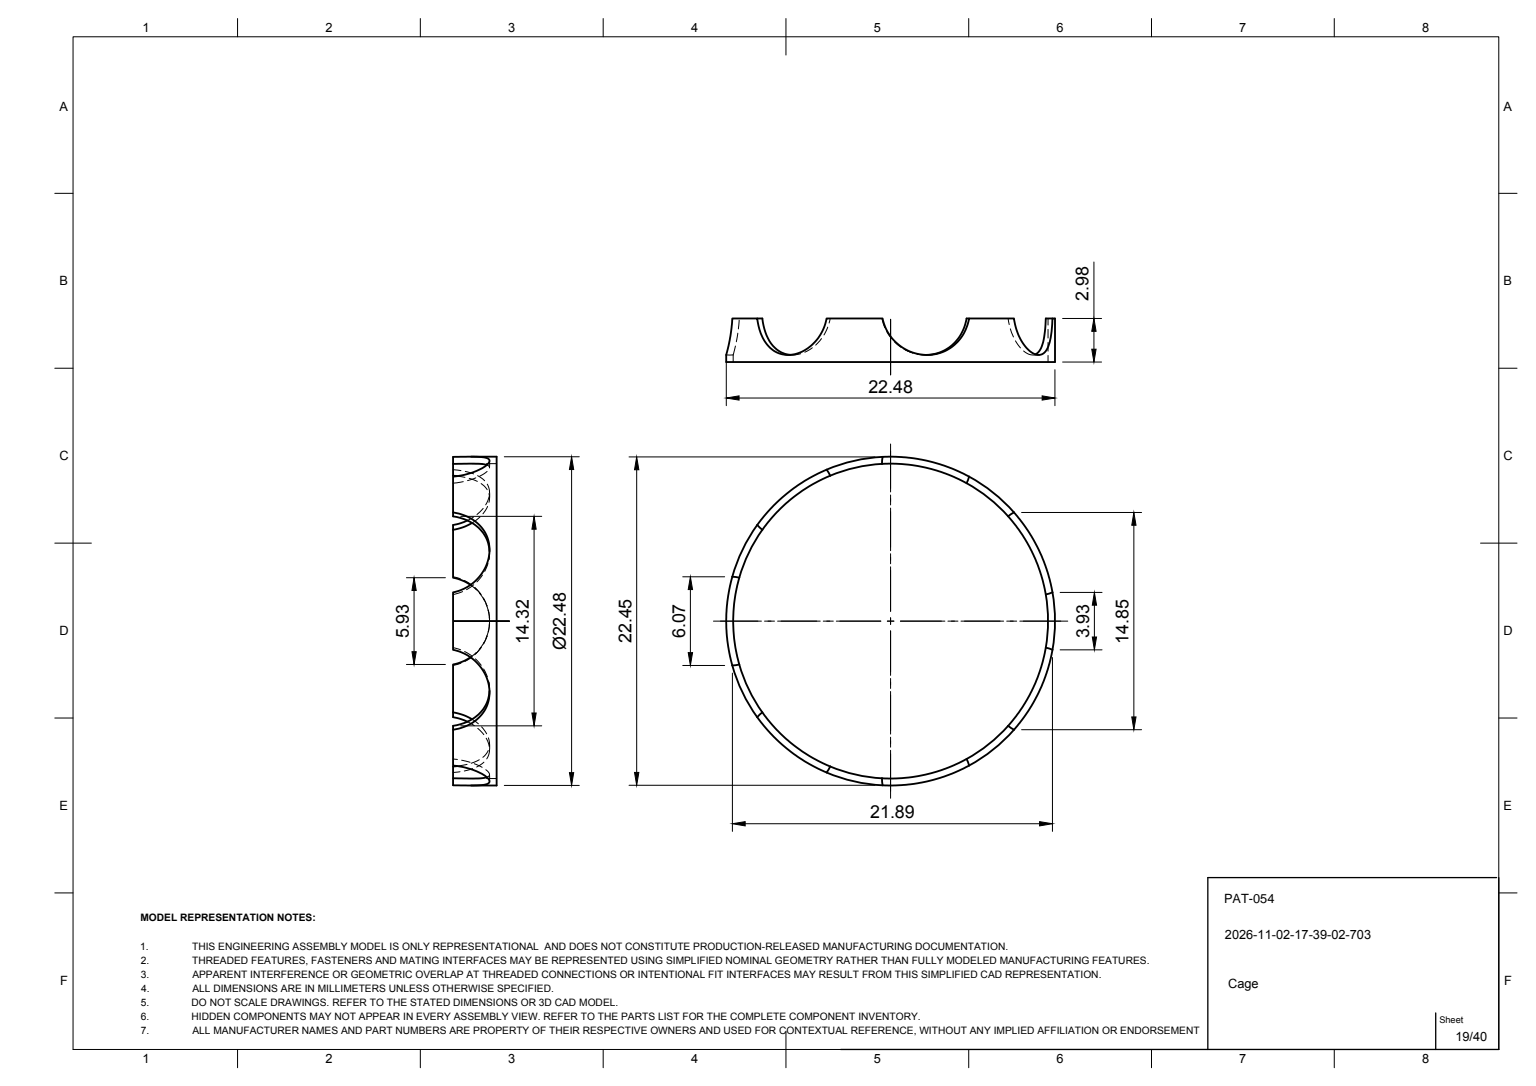
ISO-10303-21;
HEADER;
/* Generated by software containing ST-Developer
 * from STEP Tools, Inc. (www.steptools.com) 
 */

FILE_DESCRIPTION(
/* description */ ('PAT-054'),
/* implementation_level */ '2;1');

FILE_NAME(
/* name */ 'Cage.step',
/* time_stamp */ '2026-10-29T16:38:13-07:00',
/* author */ (''),
/* organization */ (''),
/* preprocessor_version */ 'ST-DEVELOPER v20.2',
/* originating_system */ 'Autodesk Translation Framework v15.17.0.0',
/* authorisation */ '');

FILE_SCHEMA (('AUTOMOTIVE_DESIGN { 1 0 10303 214 3 1 1 }'));
ENDSEC;

DATA;
#10=MECHANICAL_DESIGN_GEOMETRIC_PRESENTATION_REPRESENTATION('',(#917),#33981);
#403=B_SPLINE_CURVE_WITH_KNOTS('',3,(#19369,#19370,#19371,#19372,#19373,
#19374,#19375,#19376,#19377,#19378,#19379,#19380,#19381,#19382,#19383,#19384,
#19385,#19386,#19387,#19388,#19389,#19390),.UNSPECIFIED.,.F.,.F.,(4,2,2,
2,2,2,2,2,2,2,4),(0.0591825211272536,0.157966726598481,0.236950089897721,
0.315933453196962,0.391576304923761,0.46721915665056,0.54286200837736,0.618504860104159,
0.697488223403399,0.77647158670264,0.875255792173867),.UNSPECIFIED.);
#404=B_SPLINE_CURVE_WITH_KNOTS('',3,(#19394,#19395,#19396,#19397,#19398,
#19399,#19400,#19401,#19402,#19403,#19404,#19405,#19406,#19407,#19408,#19409,
#19410,#19411,#19412,#19413,#19414,#19415),.UNSPECIFIED.,.F.,.F.,(4,2,2,
2,2,2,2,2,2,2,4),(0.0581119756758434,0.106553146291161,0.213106292582322,
0.30849933801665,0.386091982889075,0.4636846277615,0.541277272633925,0.61886991750635,
0.714262962940678,0.820816109231839,0.869257279847157),.UNSPECIFIED.);
#405=B_SPLINE_CURVE_WITH_KNOTS('',3,(#19421,#19422,#19423,#19424,#19425,
#19426,#19427,#19428,#19429,#19430,#19431,#19432,#19433,#19434,#19435,#19436,
#19437,#19438,#19439,#19440,#19441,#19442),.UNSPECIFIED.,.F.,.F.,(4,2,2,
2,2,2,2,2,2,2,4),(0.0581119756758434,0.106553146291161,0.213106292582322,
0.30849933801665,0.386091982889075,0.4636846277615,0.541277272633925,0.61886991750635,
0.714262962940679,0.820816109231839,0.869257279847157),.UNSPECIFIED.);
#406=B_SPLINE_CURVE_WITH_KNOTS('',3,(#19446,#19447,#19448,#19449,#19450,
#19451,#19452,#19453,#19454,#19455,#19456,#19457,#19458,#19459,#19460,#19461,
#19462,#19463,#19464,#19465,#19466,#19467),.UNSPECIFIED.,.F.,.F.,(4,2,2,
2,2,2,2,2,2,2,4),(0.0581119756758433,0.106553146291161,0.213106292582322,
0.308499338016649,0.386091982889075,0.4636846277615,0.541277272633925,0.61886991750635,
0.714262962940678,0.820816109231839,0.869257279847157),.UNSPECIFIED.);
#407=B_SPLINE_CURVE_WITH_KNOTS('',3,(#19476,#19477,#19478,#19479,#19480,
#19481,#19482,#19483,#19484,#19485,#19486,#19487,#19488,#19489,#19490,#19491,
#19492,#19493,#19494,#19495,#19496,#19497),.UNSPECIFIED.,.F.,.F.,(4,2,2,
2,2,2,2,2,2,2,4),(0.0581119756758433,0.106553146291161,0.213106292582322,
0.30849933801665,0.386091982889075,0.4636846277615,0.541277272633925,0.61886991750635,
0.714262962940678,0.820816109231839,0.869257279847157),.UNSPECIFIED.);
#408=B_SPLINE_CURVE_WITH_KNOTS('',3,(#19501,#19502,#19503,#19504,#19505,
#19506,#19507,#19508,#19509,#19510,#19511,#19512,#19513,#19514,#19515,#19516,
#19517,#19518,#19519,#19520,#19521,#19522),.UNSPECIFIED.,.F.,.F.,(4,2,2,
2,2,2,2,2,2,2,4),(0.0581119756758434,0.106553146291161,0.213106292582322,
0.30849933801665,0.386091982889075,0.4636846277615,0.541277272633925,0.61886991750635,
0.714262962940678,0.820816109231839,0.869257279847157),.UNSPECIFIED.);
#409=B_SPLINE_CURVE_WITH_KNOTS('',3,(#19526,#19527,#19528,#19529,#19530,
#19531,#19532,#19533,#19534,#19535,#19536,#19537,#19538,#19539,#19540,#19541,
#19542,#19543,#19544,#19545,#19546,#19547),.UNSPECIFIED.,.F.,.F.,(4,2,2,
2,2,2,2,2,2,2,4),(0.0581119756758434,0.106553146291161,0.213106292582322,
0.30849933801665,0.386091982889075,0.4636846277615,0.541277272633925,0.61886991750635,
0.714262962940678,0.820816109231839,0.869257279847157),.UNSPECIFIED.);
#410=B_SPLINE_CURVE_WITH_KNOTS('',3,(#19551,#19552,#19553,#19554,#19555,
#19556,#19557,#19558,#19559,#19560,#19561,#19562,#19563,#19564,#19565,#19566,
#19567,#19568,#19569,#19570,#19571,#19572),.UNSPECIFIED.,.F.,.F.,(4,2,2,
2,2,2,2,2,2,2,4),(0.0581119756758433,0.106553146291161,0.213106292582322,
0.30849933801665,0.386091982889075,0.4636846277615,0.541277272633925,0.61886991750635,
0.714262962940678,0.820816109231839,0.869257279847157),.UNSPECIFIED.);
#411=B_SPLINE_CURVE_WITH_KNOTS('',3,(#19580,#19581,#19582,#19583,#19584,
#19585,#19586,#19587,#19588,#19589,#19590,#19591,#19592,#19593,#19594,#19595,
#19596,#19597,#19598,#19599,#19600,#19601),.UNSPECIFIED.,.F.,.F.,(4,2,2,
2,2,2,2,2,2,2,4),(0.0591825211272536,0.157966726598481,0.236950089897721,
0.315933453196962,0.391576304923761,0.467219156650561,0.54286200837736,
0.618504860104159,0.697488223403399,0.77647158670264,0.875255792173867),
 .UNSPECIFIED.);
#412=B_SPLINE_CURVE_WITH_KNOTS('',3,(#19609,#19610,#19611,#19612,#19613,
#19614,#19615,#19616,#19617,#19618,#19619,#19620,#19621,#19622,#19623,#19624,
#19625,#19626,#19627,#19628,#19629,#19630),.UNSPECIFIED.,.F.,.F.,(4,2,2,
2,2,2,2,2,2,2,4),(0.0591825211272536,0.157966726598481,0.236950089897722,
0.315933453196962,0.391576304923761,0.467219156650561,0.54286200837736,
0.618504860104159,0.697488223403399,0.77647158670264,0.875255792173867),
 .UNSPECIFIED.);
#413=B_SPLINE_CURVE_WITH_KNOTS('',3,(#19640,#19641,#19642,#19643,#19644,
#19645,#19646,#19647,#19648,#19649,#19650,#19651,#19652,#19653,#19654,#19655,
#19656,#19657,#19658,#19659,#19660,#19661),.UNSPECIFIED.,.F.,.F.,(4,2,2,
2,2,2,2,2,2,2,4),(0.0591825211272536,0.157966726598481,0.236950089897721,
0.315933453196962,0.391576304923761,0.46721915665056,0.54286200837736,0.618504860104159,
0.697488223403399,0.77647158670264,0.875255792173867),.UNSPECIFIED.);
#414=B_SPLINE_CURVE_WITH_KNOTS('',3,(#19669,#19670,#19671,#19672,#19673,
#19674,#19675,#19676,#19677,#19678,#19679,#19680,#19681,#19682,#19683,#19684,
#19685,#19686,#19687,#19688,#19689,#19690),.UNSPECIFIED.,.F.,.F.,(4,2,2,
2,2,2,2,2,2,2,4),(0.0591825211272536,0.157966726598481,0.236950089897721,
0.315933453196962,0.391576304923761,0.46721915665056,0.542862008377359,
0.618504860104159,0.697488223403399,0.776471586702639,0.875255792173867),
 .UNSPECIFIED.);
#415=B_SPLINE_CURVE_WITH_KNOTS('',3,(#19698,#19699,#19700,#19701,#19702,
#19703,#19704,#19705,#19706,#19707,#19708,#19709,#19710,#19711,#19712,#19713,
#19714,#19715,#19716,#19717,#19718,#19719),.UNSPECIFIED.,.F.,.F.,(4,2,2,
2,2,2,2,2,2,2,4),(0.0591825211272536,0.157966726598481,0.236950089897721,
0.315933453196962,0.391576304923761,0.46721915665056,0.54286200837736,0.618504860104159,
0.697488223403399,0.77647158670264,0.875255792173867),.UNSPECIFIED.);
#416=B_SPLINE_CURVE_WITH_KNOTS('',3,(#19728,#19729,#19730,#19731,#19732,
#19733,#19734,#19735,#19736,#19737,#19738,#19739,#19740,#19741,#19742,#19743,
#19744,#19745,#19746,#19747,#19748,#19749),.UNSPECIFIED.,.F.,.F.,(4,2,2,
2,2,2,2,2,2,2,4),(0.0591825211272536,0.157966726598481,0.236950089897721,
0.315933453196962,0.391576304923761,0.46721915665056,0.542862008377359,
0.618504860104159,0.697488223403399,0.776471586702639,0.875255792173867),
 .UNSPECIFIED.);
#754=SPHERICAL_SURFACE('',#13928,0.309556);
#755=SPHERICAL_SURFACE('',#13944,0.309556);
#756=SPHERICAL_SURFACE('',#13949,0.309556);
#757=SPHERICAL_SURFACE('',#13955,0.309556);
#758=SPHERICAL_SURFACE('',#13960,0.309556);
#759=SPHERICAL_SURFACE('',#13965,0.309556);
#760=SPHERICAL_SURFACE('',#13973,0.309556);
#823=SHAPE_REPRESENTATION_RELATIONSHIP('SRR','None',#34197,#867);
#867=ADVANCED_BREP_SHAPE_REPRESENTATION('',(#976),#33945);
#917=STYLED_ITEM('',(#34517),#976);
#976=MANIFOLD_SOLID_BREP('Continuous crown cage',#13028);
#1132=FACE_BOUND('',#2610,.T.);
#1315=PLANE('',#13941);
#1316=PLANE('',#13946);
#1317=PLANE('',#13951);
#1318=PLANE('',#13957);
#1319=PLANE('',#13962);
#1320=PLANE('',#13971);
#1321=PLANE('',#13975);
#1322=PLANE('',#13976);
#1751=FACE_OUTER_BOUND('',#2594,.T.);
#1752=FACE_OUTER_BOUND('',#2595,.T.);
#1753=FACE_OUTER_BOUND('',#2596,.T.);
#1754=FACE_OUTER_BOUND('',#2597,.T.);
#1755=FACE_OUTER_BOUND('',#2598,.T.);
#1756=FACE_OUTER_BOUND('',#2599,.T.);
#1757=FACE_OUTER_BOUND('',#2600,.T.);
#1758=FACE_OUTER_BOUND('',#2601,.T.);
#1759=FACE_OUTER_BOUND('',#2602,.T.);
#1760=FACE_OUTER_BOUND('',#2603,.T.);
#1761=FACE_OUTER_BOUND('',#2604,.T.);
#1762=FACE_OUTER_BOUND('',#2605,.T.);
#1763=FACE_OUTER_BOUND('',#2606,.T.);
#1764=FACE_OUTER_BOUND('',#2607,.T.);
#1765=FACE_OUTER_BOUND('',#2608,.T.);
#1766=FACE_OUTER_BOUND('',#2609,.T.);
#1767=FACE_OUTER_BOUND('',#2611,.T.);
#2594=EDGE_LOOP('',(#9305,#9306,#9307,#9308));
#2595=EDGE_LOOP('',(#9309,#9310,#9311,#9312,#9313,#9314,#9315,#9316,#9317,
#9318,#9319,#9320,#9321,#9322,#9323,#9324,#9325,#9326));
#2596=EDGE_LOOP('',(#9327,#9328,#9329,#9330));
#2597=EDGE_LOOP('',(#9331,#9332,#9333,#9334));
#2598=EDGE_LOOP('',(#9335,#9336,#9337,#9338));
#2599=EDGE_LOOP('',(#9339,#9340,#9341,#9342));
#2600=EDGE_LOOP('',(#9343,#9344,#9345,#9346,#9347,#9348));
#2601=EDGE_LOOP('',(#9349,#9350,#9351,#9352));
#2602=EDGE_LOOP('',(#9353,#9354,#9355,#9356));
#2603=EDGE_LOOP('',(#9357,#9358,#9359,#9360));
#2604=EDGE_LOOP('',(#9361,#9362,#9363,#9364));
#2605=EDGE_LOOP('',(#9365,#9366,#9367,#9368));
#2606=EDGE_LOOP('',(#9369,#9370,#9371,#9372,#9373,#9374,#9375,#9376,#9377,
#9378,#9379,#9380,#9381,#9382,#9383,#9384,#9385,#9386));
#2607=EDGE_LOOP('',(#9387,#9388,#9389,#9390));
#2608=EDGE_LOOP('',(#9391,#9392,#9393,#9394));
#2609=EDGE_LOOP('',(#9395));
#2610=EDGE_LOOP('',(#9396));
#2611=EDGE_LOOP('',(#9397,#9398,#9399,#9400));
#3468=LINE('',#19471,#4402);
#3469=LINE('',#19724,#4403);
#4402=VECTOR('',#15873,1.123812);
#4403=VECTOR('',#15942,1.076188);
#5282=CIRCLE('',#13929,0.303778037777585);
#5283=CIRCLE('',#13930,0.303778037777585);
#5284=CIRCLE('',#13932,1.123812);
#5285=CIRCLE('',#13933,1.123812);
#5286=CIRCLE('',#13934,1.123812);
#5287=CIRCLE('',#13935,1.123812);
#5288=CIRCLE('',#13936,1.123812);
#5289=CIRCLE('',#13937,1.123812);
#5290=CIRCLE('',#13938,1.123812);
#5291=CIRCLE('',#13939,1.123812);
#5292=CIRCLE('',#13940,1.123812);
#5293=CIRCLE('',#13942,1.076188);
#5294=CIRCLE('',#13943,0.303778037777585);
#5295=CIRCLE('',#13945,0.303778037777585);
#5296=CIRCLE('',#13947,1.076188);
#5297=CIRCLE('',#13948,0.303778037777585);
#5298=CIRCLE('',#13950,0.303778037777585);
#5299=CIRCLE('',#13952,1.076188);
#5300=CIRCLE('',#13953,1.076188);
#5301=CIRCLE('',#13954,0.303778037777585);
#5302=CIRCLE('',#13956,0.303778037777585);
#5303=CIRCLE('',#13958,1.076188);
#5304=CIRCLE('',#13959,0.303778037777585);
#5305=CIRCLE('',#13961,0.303778037777585);
#5306=CIRCLE('',#13963,1.076188);
#5307=CIRCLE('',#13964,0.303778037777585);
#5308=CIRCLE('',#13966,0.303778037777585);
#5309=CIRCLE('',#13968,1.076188);
#5310=CIRCLE('',#13969,1.076188);
#5311=CIRCLE('',#13970,1.076188);
#5312=CIRCLE('',#13972,0.303778037777585);
#5313=CIRCLE('',#13974,0.303778037777585);
#5850=VERTEX_POINT('',#19367);
#5851=VERTEX_POINT('',#19368);
#5852=VERTEX_POINT('',#19391);
#5853=VERTEX_POINT('',#19393);
#5854=VERTEX_POINT('',#19418);
#5855=VERTEX_POINT('',#19420);
#5856=VERTEX_POINT('',#19443);
#5857=VERTEX_POINT('',#19445);
#5858=VERTEX_POINT('',#19468);
#5859=VERTEX_POINT('',#19470);
#5860=VERTEX_POINT('',#19473);
#5861=VERTEX_POINT('',#19475);
#5862=VERTEX_POINT('',#19498);
#5863=VERTEX_POINT('',#19500);
#5864=VERTEX_POINT('',#19523);
#5865=VERTEX_POINT('',#19525);
#5866=VERTEX_POINT('',#19548);
#5867=VERTEX_POINT('',#19550);
#5868=VERTEX_POINT('',#19575);
#5869=VERTEX_POINT('',#19579);
#5870=VERTEX_POINT('',#19604);
#5871=VERTEX_POINT('',#19608);
#5872=VERTEX_POINT('',#19633);
#5873=VERTEX_POINT('',#19635);
#5874=VERTEX_POINT('',#19639);
#5875=VERTEX_POINT('',#19664);
#5876=VERTEX_POINT('',#19668);
#5877=VERTEX_POINT('',#19693);
#5878=VERTEX_POINT('',#19697);
#5879=VERTEX_POINT('',#19722);
#5880=VERTEX_POINT('',#19725);
#5881=VERTEX_POINT('',#19727);
#7152=EDGE_CURVE('',#5850,#5851,#403,.T.);
#7153=EDGE_CURVE('',#5852,#5850,#5282,.T.);
#7154=EDGE_CURVE('',#5853,#5852,#404,.T.);
#7155=EDGE_CURVE('',#5851,#5853,#5283,.T.);
#7156=EDGE_CURVE('',#5854,#5852,#5284,.T.);
#7157=EDGE_CURVE('',#5854,#5855,#405,.T.);
#7158=EDGE_CURVE('',#5856,#5855,#5285,.T.);
#7159=EDGE_CURVE('',#5856,#5857,#406,.T.);
#7160=EDGE_CURVE('',#5858,#5857,#5286,.T.);
#7161=EDGE_CURVE('',#5858,#5859,#3468,.T.);
#7162=EDGE_CURVE('',#5859,#5859,#5287,.T.);
#7163=EDGE_CURVE('',#5860,#5858,#5288,.T.);
#7164=EDGE_CURVE('',#5860,#5861,#407,.T.);
#7165=EDGE_CURVE('',#5862,#5861,#5289,.T.);
#7166=EDGE_CURVE('',#5862,#5863,#408,.T.);
#7167=EDGE_CURVE('',#5864,#5863,#5290,.T.);
#7168=EDGE_CURVE('',#5864,#5865,#409,.T.);
#7169=EDGE_CURVE('',#5866,#5865,#5291,.T.);
#7170=EDGE_CURVE('',#5866,#5867,#410,.T.);
#7171=EDGE_CURVE('',#5853,#5867,#5292,.T.);
#7172=EDGE_CURVE('',#5850,#5868,#5293,.T.);
#7173=EDGE_CURVE('',#5868,#5854,#5294,.T.);
#7174=EDGE_CURVE('',#5869,#5868,#411,.T.);
#7175=EDGE_CURVE('',#5855,#5869,#5295,.T.);
#7176=EDGE_CURVE('',#5869,#5870,#5296,.T.);
#7177=EDGE_CURVE('',#5870,#5856,#5297,.T.);
#7178=EDGE_CURVE('',#5871,#5870,#412,.T.);
#7179=EDGE_CURVE('',#5857,#5871,#5298,.T.);
#7180=EDGE_CURVE('',#5871,#5872,#5299,.T.);
#7181=EDGE_CURVE('',#5872,#5873,#5300,.T.);
#7182=EDGE_CURVE('',#5873,#5860,#5301,.T.);
#7183=EDGE_CURVE('',#5874,#5873,#413,.T.);
#7184=EDGE_CURVE('',#5861,#5874,#5302,.T.);
#7185=EDGE_CURVE('',#5874,#5875,#5303,.T.);
#7186=EDGE_CURVE('',#5875,#5862,#5304,.T.);
#7187=EDGE_CURVE('',#5876,#5875,#414,.T.);
#7188=EDGE_CURVE('',#5863,#5876,#5305,.T.);
#7189=EDGE_CURVE('',#5876,#5877,#5306,.T.);
#7190=EDGE_CURVE('',#5877,#5864,#5307,.T.);
#7191=EDGE_CURVE('',#5878,#5877,#415,.T.);
#7192=EDGE_CURVE('',#5865,#5878,#5308,.T.);
#7193=EDGE_CURVE('',#5879,#5879,#5309,.T.);
#7194=EDGE_CURVE('',#5879,#5872,#3469,.T.);
#7195=EDGE_CURVE('',#5880,#5851,#5310,.T.);
#7196=EDGE_CURVE('',#5880,#5881,#416,.T.);
#7197=EDGE_CURVE('',#5878,#5881,#5311,.T.);
#7198=EDGE_CURVE('',#5867,#5880,#5312,.T.);
#7199=EDGE_CURVE('',#5881,#5866,#5313,.T.);
#9305=ORIENTED_EDGE('',*,*,#7152,.F.);
#9306=ORIENTED_EDGE('',*,*,#7153,.F.);
#9307=ORIENTED_EDGE('',*,*,#7154,.F.);
#9308=ORIENTED_EDGE('',*,*,#7155,.F.);
#9309=ORIENTED_EDGE('',*,*,#7154,.T.);
#9310=ORIENTED_EDGE('',*,*,#7156,.F.);
#9311=ORIENTED_EDGE('',*,*,#7157,.T.);
#9312=ORIENTED_EDGE('',*,*,#7158,.F.);
#9313=ORIENTED_EDGE('',*,*,#7159,.T.);
#9314=ORIENTED_EDGE('',*,*,#7160,.F.);
#9315=ORIENTED_EDGE('',*,*,#7161,.T.);
#9316=ORIENTED_EDGE('',*,*,#7162,.F.);
#9317=ORIENTED_EDGE('',*,*,#7161,.F.);
#9318=ORIENTED_EDGE('',*,*,#7163,.F.);
#9319=ORIENTED_EDGE('',*,*,#7164,.T.);
#9320=ORIENTED_EDGE('',*,*,#7165,.F.);
#9321=ORIENTED_EDGE('',*,*,#7166,.T.);
#9322=ORIENTED_EDGE('',*,*,#7167,.F.);
#9323=ORIENTED_EDGE('',*,*,#7168,.T.);
#9324=ORIENTED_EDGE('',*,*,#7169,.F.);
#9325=ORIENTED_EDGE('',*,*,#7170,.T.);
#9326=ORIENTED_EDGE('',*,*,#7171,.F.);
#9327=ORIENTED_EDGE('',*,*,#7153,.T.);
#9328=ORIENTED_EDGE('',*,*,#7172,.T.);
#9329=ORIENTED_EDGE('',*,*,#7173,.T.);
#9330=ORIENTED_EDGE('',*,*,#7156,.T.);
#9331=ORIENTED_EDGE('',*,*,#7174,.F.);
#9332=ORIENTED_EDGE('',*,*,#7175,.F.);
#9333=ORIENTED_EDGE('',*,*,#7157,.F.);
#9334=ORIENTED_EDGE('',*,*,#7173,.F.);
#9335=ORIENTED_EDGE('',*,*,#7175,.T.);
#9336=ORIENTED_EDGE('',*,*,#7176,.T.);
#9337=ORIENTED_EDGE('',*,*,#7177,.T.);
#9338=ORIENTED_EDGE('',*,*,#7158,.T.);
#9339=ORIENTED_EDGE('',*,*,#7178,.F.);
#9340=ORIENTED_EDGE('',*,*,#7179,.F.);
#9341=ORIENTED_EDGE('',*,*,#7159,.F.);
#9342=ORIENTED_EDGE('',*,*,#7177,.F.);
#9343=ORIENTED_EDGE('',*,*,#7179,.T.);
#9344=ORIENTED_EDGE('',*,*,#7180,.T.);
#9345=ORIENTED_EDGE('',*,*,#7181,.T.);
#9346=ORIENTED_EDGE('',*,*,#7182,.T.);
#9347=ORIENTED_EDGE('',*,*,#7163,.T.);
#9348=ORIENTED_EDGE('',*,*,#7160,.T.);
#9349=ORIENTED_EDGE('',*,*,#7183,.F.);
#9350=ORIENTED_EDGE('',*,*,#7184,.F.);
#9351=ORIENTED_EDGE('',*,*,#7164,.F.);
#9352=ORIENTED_EDGE('',*,*,#7182,.F.);
#9353=ORIENTED_EDGE('',*,*,#7184,.T.);
#9354=ORIENTED_EDGE('',*,*,#7185,.T.);
#9355=ORIENTED_EDGE('',*,*,#7186,.T.);
#9356=ORIENTED_EDGE('',*,*,#7165,.T.);
#9357=ORIENTED_EDGE('',*,*,#7187,.F.);
#9358=ORIENTED_EDGE('',*,*,#7188,.F.);
#9359=ORIENTED_EDGE('',*,*,#7166,.F.);
#9360=ORIENTED_EDGE('',*,*,#7186,.F.);
#9361=ORIENTED_EDGE('',*,*,#7188,.T.);
#9362=ORIENTED_EDGE('',*,*,#7189,.T.);
#9363=ORIENTED_EDGE('',*,*,#7190,.T.);
#9364=ORIENTED_EDGE('',*,*,#7167,.T.);
#9365=ORIENTED_EDGE('',*,*,#7168,.F.);
#9366=ORIENTED_EDGE('',*,*,#7190,.F.);
#9367=ORIENTED_EDGE('',*,*,#7191,.F.);
#9368=ORIENTED_EDGE('',*,*,#7192,.F.);
#9369=ORIENTED_EDGE('',*,*,#7193,.F.);
#9370=ORIENTED_EDGE('',*,*,#7194,.T.);
#9371=ORIENTED_EDGE('',*,*,#7180,.F.);
#9372=ORIENTED_EDGE('',*,*,#7178,.T.);
#9373=ORIENTED_EDGE('',*,*,#7176,.F.);
#9374=ORIENTED_EDGE('',*,*,#7174,.T.);
#9375=ORIENTED_EDGE('',*,*,#7172,.F.);
#9376=ORIENTED_EDGE('',*,*,#7152,.T.);
#9377=ORIENTED_EDGE('',*,*,#7195,.F.);
#9378=ORIENTED_EDGE('',*,*,#7196,.T.);
#9379=ORIENTED_EDGE('',*,*,#7197,.F.);
#9380=ORIENTED_EDGE('',*,*,#7191,.T.);
#9381=ORIENTED_EDGE('',*,*,#7189,.F.);
#9382=ORIENTED_EDGE('',*,*,#7187,.T.);
#9383=ORIENTED_EDGE('',*,*,#7185,.F.);
#9384=ORIENTED_EDGE('',*,*,#7183,.T.);
#9385=ORIENTED_EDGE('',*,*,#7181,.F.);
#9386=ORIENTED_EDGE('',*,*,#7194,.F.);
#9387=ORIENTED_EDGE('',*,*,#7155,.T.);
#9388=ORIENTED_EDGE('',*,*,#7171,.T.);
#9389=ORIENTED_EDGE('',*,*,#7198,.T.);
#9390=ORIENTED_EDGE('',*,*,#7195,.T.);
#9391=ORIENTED_EDGE('',*,*,#7170,.F.);
#9392=ORIENTED_EDGE('',*,*,#7199,.F.);
#9393=ORIENTED_EDGE('',*,*,#7196,.F.);
#9394=ORIENTED_EDGE('',*,*,#7198,.F.);
#9395=ORIENTED_EDGE('',*,*,#7162,.T.);
#9396=ORIENTED_EDGE('',*,*,#7193,.T.);
#9397=ORIENTED_EDGE('',*,*,#7192,.T.);
#9398=ORIENTED_EDGE('',*,*,#7197,.T.);
#9399=ORIENTED_EDGE('',*,*,#7199,.T.);
#9400=ORIENTED_EDGE('',*,*,#7169,.T.);
#12055=CYLINDRICAL_SURFACE('',#13931,1.123812);
#12056=CYLINDRICAL_SURFACE('',#13967,1.076188);
#12463=ADVANCED_FACE('',(#1751),#754,.F.);
#12464=ADVANCED_FACE('',(#1752),#12055,.T.);
#12465=ADVANCED_FACE('',(#1753),#1315,.T.);
#12466=ADVANCED_FACE('',(#1754),#755,.F.);
#12467=ADVANCED_FACE('',(#1755),#1316,.T.);
#12468=ADVANCED_FACE('',(#1756),#756,.F.);
#12469=ADVANCED_FACE('',(#1757),#1317,.T.);
#12470=ADVANCED_FACE('',(#1758),#757,.F.);
#12471=ADVANCED_FACE('',(#1759),#1318,.T.);
#12472=ADVANCED_FACE('',(#1760),#758,.F.);
#12473=ADVANCED_FACE('',(#1761),#1319,.T.);
#12474=ADVANCED_FACE('',(#1762),#759,.F.);
#12475=ADVANCED_FACE('',(#1763),#12056,.F.);
#12476=ADVANCED_FACE('',(#1764),#1320,.T.);
#12477=ADVANCED_FACE('',(#1765),#760,.F.);
#12478=ADVANCED_FACE('',(#1766,#1132),#1321,.T.);
#12479=ADVANCED_FACE('',(#1767),#1322,.T.);
#13028=CLOSED_SHELL('',(#12463,#12464,#12465,#12466,#12467,#12468,#12469,
#12470,#12471,#12472,#12473,#12474,#12475,#12476,#12477,#12478,#12479));
#13927=AXIS2_PLACEMENT_3D('',#19365,#15857,#15858);
#13928=AXIS2_PLACEMENT_3D('',#19366,#15859,#15860);
#13929=AXIS2_PLACEMENT_3D('',#19392,#15861,#15862);
#13930=AXIS2_PLACEMENT_3D('',#19416,#15863,#15864);
#13931=AXIS2_PLACEMENT_3D('',#19417,#15865,#15866);
#13932=AXIS2_PLACEMENT_3D('',#19419,#15867,#15868);
#13933=AXIS2_PLACEMENT_3D('',#19444,#15869,#15870);
#13934=AXIS2_PLACEMENT_3D('',#19469,#15871,#15872);
#13935=AXIS2_PLACEMENT_3D('',#19472,#15874,#15875);
#13936=AXIS2_PLACEMENT_3D('',#19474,#15876,#15877);
#13937=AXIS2_PLACEMENT_3D('',#19499,#15878,#15879);
#13938=AXIS2_PLACEMENT_3D('',#19524,#15880,#15881);
#13939=AXIS2_PLACEMENT_3D('',#19549,#15882,#15883);
#13940=AXIS2_PLACEMENT_3D('',#19573,#15884,#15885);
#13941=AXIS2_PLACEMENT_3D('',#19574,#15886,#15887);
#13942=AXIS2_PLACEMENT_3D('',#19576,#15888,#15889);
#13943=AXIS2_PLACEMENT_3D('',#19577,#15890,#15891);
#13944=AXIS2_PLACEMENT_3D('',#19578,#15892,#15893);
#13945=AXIS2_PLACEMENT_3D('',#19602,#15894,#15895);
#13946=AXIS2_PLACEMENT_3D('',#19603,#15896,#15897);
#13947=AXIS2_PLACEMENT_3D('',#19605,#15898,#15899);
#13948=AXIS2_PLACEMENT_3D('',#19606,#15900,#15901);
#13949=AXIS2_PLACEMENT_3D('',#19607,#15902,#15903);
#13950=AXIS2_PLACEMENT_3D('',#19631,#15904,#15905);
#13951=AXIS2_PLACEMENT_3D('',#19632,#15906,#15907);
#13952=AXIS2_PLACEMENT_3D('',#19634,#15908,#15909);
#13953=AXIS2_PLACEMENT_3D('',#19636,#15910,#15911);
#13954=AXIS2_PLACEMENT_3D('',#19637,#15912,#15913);
#13955=AXIS2_PLACEMENT_3D('',#19638,#15914,#15915);
#13956=AXIS2_PLACEMENT_3D('',#19662,#15916,#15917);
#13957=AXIS2_PLACEMENT_3D('',#19663,#15918,#15919);
#13958=AXIS2_PLACEMENT_3D('',#19665,#15920,#15921);
#13959=AXIS2_PLACEMENT_3D('',#19666,#15922,#15923);
#13960=AXIS2_PLACEMENT_3D('',#19667,#15924,#15925);
#13961=AXIS2_PLACEMENT_3D('',#19691,#15926,#15927);
#13962=AXIS2_PLACEMENT_3D('',#19692,#15928,#15929);
#13963=AXIS2_PLACEMENT_3D('',#19694,#15930,#15931);
#13964=AXIS2_PLACEMENT_3D('',#19695,#15932,#15933);
#13965=AXIS2_PLACEMENT_3D('',#19696,#15934,#15935);
#13966=AXIS2_PLACEMENT_3D('',#19720,#15936,#15937);
#13967=AXIS2_PLACEMENT_3D('',#19721,#15938,#15939);
#13968=AXIS2_PLACEMENT_3D('',#19723,#15940,#15941);
#13969=AXIS2_PLACEMENT_3D('',#19726,#15943,#15944);
#13970=AXIS2_PLACEMENT_3D('',#19750,#15945,#15946);
#13971=AXIS2_PLACEMENT_3D('',#19751,#15947,#15948);
#13972=AXIS2_PLACEMENT_3D('',#19752,#15949,#15950);
#13973=AXIS2_PLACEMENT_3D('',#19753,#15951,#15952);
#13974=AXIS2_PLACEMENT_3D('',#19754,#15953,#15954);
#13975=AXIS2_PLACEMENT_3D('',#19755,#15955,#15956);
#13976=AXIS2_PLACEMENT_3D('',#19756,#15957,#15958);
#15857=DIRECTION('axis',(0.,0.,1.));
#15858=DIRECTION('refdir',(1.,0.,0.));
#15859=DIRECTION('center_axis',(0.,0.,1.));
#15860=DIRECTION('ref_axis',(1.,0.,0.));
#15861=DIRECTION('center_axis',(0.,-1.,0.));
#15862=DIRECTION('ref_axis',(0.,0.,-1.));
#15863=DIRECTION('center_axis',(0.,-1.,0.));
#15864=DIRECTION('ref_axis',(0.,0.,-1.));
#15865=DIRECTION('center_axis',(0.,1.,0.));
#15866=DIRECTION('ref_axis',(1.,0.,0.));
#15867=DIRECTION('center_axis',(0.,1.,0.));
#15868=DIRECTION('ref_axis',(1.,0.,0.));
#15869=DIRECTION('center_axis',(0.,1.,0.));
#15870=DIRECTION('ref_axis',(1.,0.,0.));
#15871=DIRECTION('center_axis',(0.,1.,0.));
#15872=DIRECTION('ref_axis',(1.,0.,0.));
#15873=DIRECTION('',(0.,-1.,0.));
#15874=DIRECTION('center_axis',(0.,-1.,0.));
#15875=DIRECTION('ref_axis',(1.,0.,0.));
#15876=DIRECTION('center_axis',(0.,1.,0.));
#15877=DIRECTION('ref_axis',(1.,0.,0.));
#15878=DIRECTION('center_axis',(0.,1.,0.));
#15879=DIRECTION('ref_axis',(1.,0.,0.));
#15880=DIRECTION('center_axis',(0.,1.,0.));
#15881=DIRECTION('ref_axis',(1.,0.,0.));
#15882=DIRECTION('center_axis',(0.,1.,0.));
#15883=DIRECTION('ref_axis',(1.,0.,0.));
#15884=DIRECTION('center_axis',(0.,1.,0.));
#15885=DIRECTION('ref_axis',(1.,0.,0.));
#15886=DIRECTION('center_axis',(0.,1.,0.));
#15887=DIRECTION('ref_axis',(1.,0.,0.));
#15888=DIRECTION('center_axis',(0.,-1.,0.));
#15889=DIRECTION('ref_axis',(1.,0.,0.));
#15890=DIRECTION('center_axis',(0.,-1.,0.));
#15891=DIRECTION('ref_axis',(0.,0.,-1.));
#15892=DIRECTION('center_axis',(8.96625347776458E-17,0.,1.));
#15893=DIRECTION('ref_axis',(1.,0.,0.));
#15894=DIRECTION('center_axis',(0.,-1.,0.));
#15895=DIRECTION('ref_axis',(0.,0.,-1.));
#15896=DIRECTION('center_axis',(0.,1.,0.));
#15897=DIRECTION('ref_axis',(1.,0.,0.));
#15898=DIRECTION('center_axis',(0.,-1.,0.));
#15899=DIRECTION('ref_axis',(1.,0.,0.));
#15900=DIRECTION('center_axis',(0.,-1.,0.));
#15901=DIRECTION('ref_axis',(0.,0.,-1.));
#15902=DIRECTION('center_axis',(0.,0.,1.));
#15903=DIRECTION('ref_axis',(1.,0.,0.));
#15904=DIRECTION('center_axis',(0.,-1.,0.));
#15905=DIRECTION('ref_axis',(0.,0.,-1.));
#15906=DIRECTION('center_axis',(0.,1.,0.));
#15907=DIRECTION('ref_axis',(1.,0.,0.));
#15908=DIRECTION('center_axis',(0.,-1.,0.));
#15909=DIRECTION('ref_axis',(1.,0.,0.));
#15910=DIRECTION('center_axis',(0.,-1.,0.));
#15911=DIRECTION('ref_axis',(1.,0.,0.));
#15912=DIRECTION('center_axis',(0.,-1.,0.));
#15913=DIRECTION('ref_axis',(0.,0.,-1.));
#15914=DIRECTION('center_axis',(0.,0.,1.));
#15915=DIRECTION('ref_axis',(1.,0.,0.));
#15916=DIRECTION('center_axis',(0.,-1.,0.));
#15917=DIRECTION('ref_axis',(0.,0.,-1.));
#15918=DIRECTION('center_axis',(0.,1.,0.));
#15919=DIRECTION('ref_axis',(1.,0.,0.));
#15920=DIRECTION('center_axis',(0.,-1.,0.));
#15921=DIRECTION('ref_axis',(1.,0.,0.));
#15922=DIRECTION('center_axis',(0.,-1.,0.));
#15923=DIRECTION('ref_axis',(0.,0.,-1.));
#15924=DIRECTION('center_axis',(8.96625347776458E-17,0.,1.));
#15925=DIRECTION('ref_axis',(1.,0.,0.));
#15926=DIRECTION('center_axis',(0.,-1.,0.));
#15927=DIRECTION('ref_axis',(0.,0.,-1.));
#15928=DIRECTION('center_axis',(0.,1.,0.));
#15929=DIRECTION('ref_axis',(1.,0.,0.));
#15930=DIRECTION('center_axis',(0.,-1.,0.));
#15931=DIRECTION('ref_axis',(1.,0.,0.));
#15932=DIRECTION('center_axis',(0.,-1.,0.));
#15933=DIRECTION('ref_axis',(0.,0.,-1.));
#15934=DIRECTION('center_axis',(0.,0.,1.));
#15935=DIRECTION('ref_axis',(1.,0.,0.));
#15936=DIRECTION('center_axis',(0.,-1.,0.));
#15937=DIRECTION('ref_axis',(0.,0.,-1.));
#15938=DIRECTION('center_axis',(0.,1.,0.));
#15939=DIRECTION('ref_axis',(1.,0.,0.));
#15940=DIRECTION('center_axis',(0.,1.,0.));
#15941=DIRECTION('ref_axis',(1.,0.,0.));
#15942=DIRECTION('',(0.,1.,0.));
#15943=DIRECTION('center_axis',(0.,-1.,0.));
#15944=DIRECTION('ref_axis',(1.,0.,0.));
#15945=DIRECTION('center_axis',(0.,-1.,0.));
#15946=DIRECTION('ref_axis',(1.,0.,0.));
#15947=DIRECTION('center_axis',(0.,1.,0.));
#15948=DIRECTION('ref_axis',(1.,0.,0.));
#15949=DIRECTION('center_axis',(0.,-1.,0.));
#15950=DIRECTION('ref_axis',(0.,0.,-1.));
#15951=DIRECTION('center_axis',(0.,0.,1.));
#15952=DIRECTION('ref_axis',(1.,0.,0.));
#15953=DIRECTION('center_axis',(0.,-1.,0.));
#15954=DIRECTION('ref_axis',(0.,0.,-1.));
#15955=DIRECTION('center_axis',(0.,-1.,0.));
#15956=DIRECTION('ref_axis',(-1.,0.,0.));
#15957=DIRECTION('center_axis',(0.,1.,0.));
#15958=DIRECTION('ref_axis',(1.,0.,0.));
#19365=CARTESIAN_POINT('',(0.,0.,0.));
#19366=CARTESIAN_POINT('Origin',(0.685838782044607,0.,0.860014630714833));
#19367=CARTESIAN_POINT('',(0.413083465285518,-0.05953,0.993751811093549));
#19368=CARTESIAN_POINT('',(0.876916659919095,-0.05953,0.623857181492959));
#19369=CARTESIAN_POINT('Ctrl Pts',(0.413083465285518,-0.05953,0.993751811093549));
#19370=CARTESIAN_POINT('Ctrl Pts',(0.419070565453383,-0.0925528133349865,
0.991263089003441));
#19371=CARTESIAN_POINT('Ctrl Pts',(0.430199341854858,-0.124911173756694,
0.986608710139579));
#19372=CARTESIAN_POINT('Ctrl Pts',(0.457978755888596,-0.177924977804098,
0.973971221090534));
#19373=CARTESIAN_POINT('Ctrl Pts',(0.473077587363685,-0.199697230012983,
0.966820759530997));
#19374=CARTESIAN_POINT('Ctrl Pts',(0.507057380724533,-0.237895043532788,
0.949440676105255));
#19375=CARTESIAN_POINT('Ctrl Pts',(0.525933334162555,-0.254319232363049,
0.939198248544428));
#19376=CARTESIAN_POINT('Ctrl Pts',(0.564362943424238,-0.28018331644634,
0.916597376014514));
#19377=CARTESIAN_POINT('Ctrl Pts',(0.585840553788742,-0.29104845371857,
0.903141581680914));
#19378=CARTESIAN_POINT('Ctrl Pts',(0.629305439856167,-0.30527573347708,
0.873412008702649));
#19379=CARTESIAN_POINT('Ctrl Pts',(0.651278921914856,-0.308638795020976,
0.857118508332695));
#19380=CARTESIAN_POINT('Ctrl Pts',(0.690705563850638,-0.308638795020976,
0.825676810575914));
#19381=CARTESIAN_POINT('Ctrl Pts',(0.711480111898423,-0.30527573347708,
0.807879894508811));
#19382=CARTESIAN_POINT('Ctrl Pts',(0.750136149454208,-0.29104845371857,
0.772120216227122));
#19383=CARTESIAN_POINT('Ctrl Pts',(0.768033796848072,-0.28018331644634,
0.754175290318038));
#19384=CARTESIAN_POINT('Ctrl Pts',(0.798619410861634,-0.254319232363049,
0.721738358858166));
#19385=CARTESIAN_POINT('Ctrl Pts',(0.812805334167529,-0.237895043532788,
0.705614819529209));
#19386=CARTESIAN_POINT('Ctrl Pts',(0.837310877969633,-0.199697230012983,
0.676354402927683));
#19387=CARTESIAN_POINT('Ctrl Pts',(0.847641868610495,-0.177924977804098,
0.663225258065736));
#19388=CARTESIAN_POINT('Ctrl Pts',(0.866144010579847,-0.124911173756694,
0.638954437806245));
#19389=CARTESIAN_POINT('Ctrl Pts',(0.873158080166742,-0.0925528133349865,
0.62914037979579));
#19390=CARTESIAN_POINT('Ctrl Pts',(0.876916659919095,-0.05953,0.623857181492959));
#19391=CARTESIAN_POINT('',(0.437601487681057,-0.05953,1.03511272300331));
#19392=CARTESIAN_POINT('Origin',(0.685838782044607,-0.05953,0.860014630714833));
#19393=CARTESIAN_POINT('',(0.911784794170997,-0.05953,0.656964154625313));
#19394=CARTESIAN_POINT('Ctrl Pts',(0.911784794170998,-0.0595300000000001,
0.656964154625312));
#19395=CARTESIAN_POINT('Ctrl Pts',(0.909827729890942,-0.0762225747374255,
0.659680317203144));
#19396=CARTESIAN_POINT('Ctrl Pts',(0.907004864562642,-0.0928409665394228,
0.663576540841106));
#19397=CARTESIAN_POINT('Ctrl Pts',(0.895234408667242,-0.144299303100741,
0.679480524217551));
#19398=CARTESIAN_POINT('Ctrl Pts',(0.882797231409153,-0.177024326825049,
0.695831250979106));
#19399=CARTESIAN_POINT('Ctrl Pts',(0.854332839576145,-0.227269801620064,
0.73042219438957));
#19400=CARTESIAN_POINT('Ctrl Pts',(0.834863020612702,-0.251265615809407,
0.752807465209441));
#19401=CARTESIAN_POINT('Ctrl Pts',(0.800439809856111,-0.279889827963178,
0.789147407129766));
#19402=CARTESIAN_POINT('Ctrl Pts',(0.781998747691871,-0.290879136862659,
0.80756613568454));
#19403=CARTESIAN_POINT('Ctrl Pts',(0.742239891936898,-0.305251990234487,
0.844254137480382));
#19404=CARTESIAN_POINT('Ctrl Pts',(0.720906778729541,-0.308638795020976,
0.862505527716294));
#19405=CARTESIAN_POINT('Ctrl Pts',(0.680463863683392,-0.308638795020976,
0.894757676234429));
#19406=CARTESIAN_POINT('Ctrl Pts',(0.657923009631182,-0.305251990234488,
0.91149460735272));
#19407=CARTESIAN_POINT('Ctrl Pts',(0.613307674922609,-0.290879136862659,
0.942092777160053));
#19408=CARTESIAN_POINT('Ctrl Pts',(0.591247219971725,-0.279889827963178,
0.955972930713954));
#19409=CARTESIAN_POINT('Ctrl Pts',(0.548158511259202,-0.251265615809407,
0.981446681891443));
#19410=CARTESIAN_POINT('Ctrl Pts',(0.522002043615455,-0.227269801620063,
0.995447160474328));
#19411=CARTESIAN_POINT('Ctrl Pts',(0.481944444320713,-0.177024326825049,
1.01550068154148));
#19412=CARTESIAN_POINT('Ctrl Pts',(0.463236132117164,-0.14429930310074,
1.0239876538093));
#19413=CARTESIAN_POINT('Ctrl Pts',(0.445111721969657,-0.0928409665394226,
1.03192403056628));
#19414=CARTESIAN_POINT('Ctrl Pts',(0.440685038163619,-0.0762225747374254,
1.03380912944435));
#19415=CARTESIAN_POINT('Ctrl Pts',(0.437601487681056,-0.05953,1.03511272300331));
#19416=CARTESIAN_POINT('Origin',(0.685838782044607,-0.05953,0.860014630714833));
#19417=CARTESIAN_POINT('Origin',(0.,-0.208355,0.));
#19418=CARTESIAN_POINT('',(0.0548532617164168,-0.05953,1.12247250791415));
#19419=CARTESIAN_POINT('Origin',(0.,-0.05953,0.));
#19420=CARTESIAN_POINT('',(-0.536443649899848,-0.05953,0.987512846410683));
#19421=CARTESIAN_POINT('Ctrl Pts',(0.0548532617164173,-0.0595300000000001,
1.12247250791414));
#19422=CARTESIAN_POINT('Ctrl Pts',(0.05150947068137,-0.0762225747374254,
1.12263591311425));
#19423=CARTESIAN_POINT('Ctrl Pts',(0.0467032526342597,-0.0928409665394227,
1.12285816383385));
#19424=CARTESIAN_POINT('Ctrl Pts',(0.0269302585198975,-0.144299303100741,
1.12357162229597));
#19425=CARTESIAN_POINT('Ctrl Pts',(0.006392292392153,-0.177024326825049,
1.12404235695137));
#19426=CARTESIAN_POINT('Ctrl Pts',(-0.0383992541984087,-0.227269801620063,
1.12335509974011));
#19427=CARTESIAN_POINT('Ctrl Pts',(-0.0680399972366993,-0.251265615809407,
1.12208997038458));
#19428=CARTESIAN_POINT('Ctrl Pts',(-0.117914228755037,-0.279889827963178,
1.1178344036749));
#19429=CARTESIAN_POINT('Ctrl Pts',(-0.14381238480104,-0.290879136862659,
1.11490049012186));
#19430=CARTESIAN_POINT('Ctrl Pts',(-0.19728546073067,-0.305251990234488,
1.10669035995599));
#19431=CARTESIAN_POINT('Ctrl Pts',(-0.224855950742601,-0.308638795020976,
1.10139101611326));
#19432=CARTESIAN_POINT('Ctrl Pts',(-0.275287440920027,-0.308638795020976,
1.0898803575765));
#19433=CARTESIAN_POINT('Ctrl Pts',(-0.302426893214945,-0.305251990234488,
1.08269251410343));
#19434=CARTESIAN_POINT('Ctrl Pts',(-0.35416671187353,-0.290879136862659,
1.06688848765783));
#19435=CARTESIAN_POINT('Ctrl Pts',(-0.3787731215897,-0.279889827963178,
1.05829506364875));
#19436=CARTESIAN_POINT('Ctrl Pts',(-0.425554672694338,-0.251265615809407,
1.04048957871266));
#19437=CARTESIAN_POINT('Ctrl Pts',(-0.452808978448581,-0.227269801620063,
1.02876878445619));
#19438=CARTESIAN_POINT('Ctrl Pts',(-0.493462957200432,-0.177024326825049,
1.0099536580922));
#19439=CARTESIAN_POINT('Ctrl Pts',(-0.511762781179148,-0.14429930310074,
1.00061845128527));
#19440=CARTESIAN_POINT('Ctrl Pts',(-0.529268075276157,-0.0928409665394226,
0.991396466802468));
#19441=CARTESIAN_POINT('Ctrl Pts',(-0.533501897135713,-0.0762225747374254,
0.989110885965947));
#19442=CARTESIAN_POINT('Ctrl Pts',(-0.536443649899848,-0.0595300000000001,
0.987512846410683));
#19443=CARTESIAN_POINT('',(-0.843383895613249,-0.05953,0.742736168477219));
#19444=CARTESIAN_POINT('Origin',(0.,-0.05953,0.));
#19445=CARTESIAN_POINT('',(-1.10653577764992,-0.05953,0.196295654879792));
#19446=CARTESIAN_POINT('Ctrl Pts',(-0.843383895613249,-0.0595300000000001,
0.742736168477219));
#19447=CARTESIAN_POINT('Ctrl Pts',(-0.84559647055299,-0.0762225747374255,
0.740223768851062));
#19448=CARTESIAN_POINT('Ctrl Pts',(-0.848766861100456,-0.0928409665394227,
0.736604687327351));
#19449=CARTESIAN_POINT('Ctrl Pts',(-0.861652925570091,-0.144299303100741,
0.721590372101268));
#19450=CARTESIAN_POINT('Ctrl Pts',(-0.87482617317514,-0.177024326825049,
0.705826641853758));
#19451=CARTESIAN_POINT('Ctrl Pts',(-0.902215926359523,-0.227269801620063,
0.670378702718353));
#19452=CARTESIAN_POINT('Ctrl Pts',(-0.919707509403859,-0.251265615809407,
0.646415841396062));
#19453=CARTESIAN_POINT('Ctrl Pts',(-0.947476448101718,-0.279889827963178,
0.604769294586516));
#19454=CARTESIAN_POINT('Ctrl Pts',(-0.961329858300736,-0.290879136862659,
0.582692035672022));
#19455=CARTESIAN_POINT('Ctrl Pts',(-0.988250837578047,-0.305251990234488,
0.535766169015486));
#19456=CARTESIAN_POINT('Ctrl Pts',(-1.00129756308006,-0.308638795020976,
0.510906605094603));
#19457=CARTESIAN_POINT('Ctrl Pts',(-1.02374168767024,-0.308638795020976,
0.46430090015576));
#19458=CARTESIAN_POINT('Ctrl Pts',(-1.03504317708586,-0.305251990234488,
0.438600874831839));
#19459=CARTESIAN_POINT('Ctrl Pts',(-1.05494634094458,-0.290879136862659,
0.388295406390235));
#19460=CARTESIAN_POINT('Ctrl Pts',(-1.06356957703048,-0.279889827963178,
0.363699428370917));
#19461=CARTESIAN_POINT('Ctrl Pts',(-1.0788165083757,-0.251265615809407,
0.316022600643821));
#19462=CARTESIAN_POINT('Ctrl Pts',(-1.08664560412098,-0.227269801620063,
0.287406530683752));
#19463=CARTESIAN_POINT('Ctrl Pts',(-1.09728268713976,-0.177024326825049,
0.243890930799337));
#19464=CARTESIAN_POINT('Ctrl Pts',(-1.10139388218929,-0.144299303100741,
0.22376314604679));
#19465=CARTESIAN_POINT('Ctrl Pts',(-1.10509821673782,-0.0928409665394227,
0.204327142733961));
#19466=CARTESIAN_POINT('Ctrl Pts',(-1.10595102243643,-0.0762225747374254,
0.199591971170104));
#19467=CARTESIAN_POINT('Ctrl Pts',(-1.10653577764992,-0.0595300000000001,
0.196295654879792));
#19468=CARTESIAN_POINT('',(-1.123812,-0.05953,1.37627276864339E-16));
#19469=CARTESIAN_POINT('Origin',(0.,-0.05953,0.));
#19470=CARTESIAN_POINT('',(-1.123812,-0.35718,1.37627276864339E-16));
#19471=CARTESIAN_POINT('',(-1.123812,-0.208355,1.37627276864339E-16));
#19472=CARTESIAN_POINT('Origin',(0.,-0.35718,0.));
#19473=CARTESIAN_POINT('',(-1.10653577764992,-0.05953,-0.196295654879793));
#19474=CARTESIAN_POINT('Origin',(0.,-0.05953,0.));
#19475=CARTESIAN_POINT('',(-0.843383895613249,-0.05953,-0.742736168477219));
#19476=CARTESIAN_POINT('Ctrl Pts',(-1.10653577764992,-0.0595300000000001,
-0.196295654879792));
#19477=CARTESIAN_POINT('Ctrl Pts',(-1.10595102243643,-0.0762225747374255,
-0.199591971170104));
#19478=CARTESIAN_POINT('Ctrl Pts',(-1.10509821673782,-0.0928409665394228,
-0.204327142733962));
#19479=CARTESIAN_POINT('Ctrl Pts',(-1.10139388218929,-0.144299303100741,
-0.22376314604679));
#19480=CARTESIAN_POINT('Ctrl Pts',(-1.09728268713976,-0.177024326825049,
-0.243890930799338));
#19481=CARTESIAN_POINT('Ctrl Pts',(-1.08664560412098,-0.227269801620063,
-0.287406530683753));
#19482=CARTESIAN_POINT('Ctrl Pts',(-1.0788165083757,-0.251265615809407,
-0.316022600643821));
#19483=CARTESIAN_POINT('Ctrl Pts',(-1.06356957703048,-0.279889827963178,
-0.363699428370918));
#19484=CARTESIAN_POINT('Ctrl Pts',(-1.05494634094458,-0.290879136862659,
-0.388295406390235));
#19485=CARTESIAN_POINT('Ctrl Pts',(-1.03504317708586,-0.305251990234488,
-0.438600874831839));
#19486=CARTESIAN_POINT('Ctrl Pts',(-1.02374168767024,-0.308638795020976,
-0.46430090015576));
#19487=CARTESIAN_POINT('Ctrl Pts',(-1.00129756308006,-0.308638795020976,
-0.510906605094603));
#19488=CARTESIAN_POINT('Ctrl Pts',(-0.988250837578047,-0.305251990234488,
-0.535766169015486));
#19489=CARTESIAN_POINT('Ctrl Pts',(-0.961329858300736,-0.290879136862659,
-0.582692035672022));
#19490=CARTESIAN_POINT('Ctrl Pts',(-0.947476448101718,-0.279889827963178,
-0.604769294586516));
#19491=CARTESIAN_POINT('Ctrl Pts',(-0.919707509403859,-0.251265615809407,
-0.646415841396062));
#19492=CARTESIAN_POINT('Ctrl Pts',(-0.902215926359523,-0.227269801620064,
-0.670378702718353));
#19493=CARTESIAN_POINT('Ctrl Pts',(-0.87482617317514,-0.177024326825049,
-0.705826641853758));
#19494=CARTESIAN_POINT('Ctrl Pts',(-0.861652925570091,-0.144299303100741,
-0.721590372101268));
#19495=CARTESIAN_POINT('Ctrl Pts',(-0.848766861100456,-0.0928409665394229,
-0.736604687327351));
#19496=CARTESIAN_POINT('Ctrl Pts',(-0.84559647055299,-0.0762225747374255,
-0.740223768851063));
#19497=CARTESIAN_POINT('Ctrl Pts',(-0.843383895613249,-0.0595300000000001,
-0.742736168477219));
#19498=CARTESIAN_POINT('',(-0.536443649899847,-0.05953,-0.987512846410683));
#19499=CARTESIAN_POINT('Origin',(0.,-0.05953,0.));
#19500=CARTESIAN_POINT('',(0.0548532617164172,-0.05953,-1.12247250791415));
#19501=CARTESIAN_POINT('Ctrl Pts',(-0.536443649899848,-0.0595300000000001,
-0.987512846410683));
#19502=CARTESIAN_POINT('Ctrl Pts',(-0.533501897135712,-0.0762225747374254,
-0.989110885965947));
#19503=CARTESIAN_POINT('Ctrl Pts',(-0.529268075276156,-0.0928409665394227,
-0.991396466802469));
#19504=CARTESIAN_POINT('Ctrl Pts',(-0.511762781179147,-0.144299303100741,
-1.00061845128527));
#19505=CARTESIAN_POINT('Ctrl Pts',(-0.493462957200432,-0.177024326825049,
-1.0099536580922));
#19506=CARTESIAN_POINT('Ctrl Pts',(-0.45280897844858,-0.227269801620063,
-1.02876878445619));
#19507=CARTESIAN_POINT('Ctrl Pts',(-0.425554672694337,-0.251265615809407,
-1.04048957871266));
#19508=CARTESIAN_POINT('Ctrl Pts',(-0.3787731215897,-0.279889827963178,
-1.05829506364875));
#19509=CARTESIAN_POINT('Ctrl Pts',(-0.354166711873529,-0.290879136862659,
-1.06688848765783));
#19510=CARTESIAN_POINT('Ctrl Pts',(-0.302426893214944,-0.305251990234488,
-1.08269251410343));
#19511=CARTESIAN_POINT('Ctrl Pts',(-0.275287440920027,-0.308638795020976,
-1.0898803575765));
#19512=CARTESIAN_POINT('Ctrl Pts',(-0.224855950742601,-0.308638795020976,
-1.10139101611326));
#19513=CARTESIAN_POINT('Ctrl Pts',(-0.19728546073067,-0.305251990234488,
-1.10669035995599));
#19514=CARTESIAN_POINT('Ctrl Pts',(-0.143812384801039,-0.290879136862659,
-1.11490049012186));
#19515=CARTESIAN_POINT('Ctrl Pts',(-0.117914228755037,-0.279889827963178,
-1.1178344036749));
#19516=CARTESIAN_POINT('Ctrl Pts',(-0.0680399972366989,-0.251265615809407,
-1.12208997038458));
#19517=CARTESIAN_POINT('Ctrl Pts',(-0.0383992541984084,-0.227269801620063,
-1.12335509974011));
#19518=CARTESIAN_POINT('Ctrl Pts',(0.00639229239215326,-0.177024326825049,
-1.12404235695137));
#19519=CARTESIAN_POINT('Ctrl Pts',(0.0269302585198977,-0.144299303100741,
-1.12357162229597));
#19520=CARTESIAN_POINT('Ctrl Pts',(0.04670325263426,-0.0928409665394228,
-1.12285816383385));
#19521=CARTESIAN_POINT('Ctrl Pts',(0.0515094706813703,-0.0762225747374255,
-1.12263591311425));
#19522=CARTESIAN_POINT('Ctrl Pts',(0.0548532617164176,-0.0595300000000001,
-1.12247250791414));
#19523=CARTESIAN_POINT('',(0.437601487681057,-0.05953,-1.03511272300331));
#19524=CARTESIAN_POINT('Origin',(0.,-0.05953,0.));
#19525=CARTESIAN_POINT('',(0.911784794170997,-0.05953,-0.656964154625313));
#19526=CARTESIAN_POINT('Ctrl Pts',(0.437601487681056,-0.0595300000000001,
-1.03511272300331));
#19527=CARTESIAN_POINT('Ctrl Pts',(0.440685038163619,-0.0762225747374255,
-1.03380912944435));
#19528=CARTESIAN_POINT('Ctrl Pts',(0.445111721969657,-0.0928409665394228,
-1.03192403056628));
#19529=CARTESIAN_POINT('Ctrl Pts',(0.463236132117164,-0.144299303100741,
-1.0239876538093));
#19530=CARTESIAN_POINT('Ctrl Pts',(0.481944444320713,-0.177024326825049,
-1.01550068154148));
#19531=CARTESIAN_POINT('Ctrl Pts',(0.522002043615455,-0.227269801620064,
-0.995447160474328));
#19532=CARTESIAN_POINT('Ctrl Pts',(0.548158511259203,-0.251265615809407,
-0.981446681891443));
#19533=CARTESIAN_POINT('Ctrl Pts',(0.591247219971725,-0.279889827963178,
-0.955972930713954));
#19534=CARTESIAN_POINT('Ctrl Pts',(0.613307674922609,-0.290879136862659,
-0.942092777160053));
#19535=CARTESIAN_POINT('Ctrl Pts',(0.657923009631182,-0.305251990234487,
-0.91149460735272));
#19536=CARTESIAN_POINT('Ctrl Pts',(0.680463863683393,-0.308638795020976,
-0.894757676234429));
#19537=CARTESIAN_POINT('Ctrl Pts',(0.720906778729542,-0.308638795020976,
-0.862505527716294));
#19538=CARTESIAN_POINT('Ctrl Pts',(0.742239891936899,-0.305251990234488,
-0.844254137480381));
#19539=CARTESIAN_POINT('Ctrl Pts',(0.781998747691872,-0.290879136862659,
-0.80756613568454));
#19540=CARTESIAN_POINT('Ctrl Pts',(0.800439809856112,-0.279889827963178,
-0.789147407129765));
#19541=CARTESIAN_POINT('Ctrl Pts',(0.834863020612702,-0.251265615809407,
-0.752807465209441));
#19542=CARTESIAN_POINT('Ctrl Pts',(0.854332839576145,-0.227269801620064,
-0.73042219438957));
#19543=CARTESIAN_POINT('Ctrl Pts',(0.882797231409153,-0.177024326825049,
-0.695831250979106));
#19544=CARTESIAN_POINT('Ctrl Pts',(0.895234408667242,-0.144299303100741,
-0.679480524217551));
#19545=CARTESIAN_POINT('Ctrl Pts',(0.907004864562642,-0.0928409665394228,
-0.663576540841106));
#19546=CARTESIAN_POINT('Ctrl Pts',(0.909827729890942,-0.0762225747374256,
-0.659680317203144));
#19547=CARTESIAN_POINT('Ctrl Pts',(0.911784794170998,-0.0595300000000001,
-0.656964154625312));
#19548=CARTESIAN_POINT('',(1.08212377959455,-0.05953,-0.303251606722892));
#19549=CARTESIAN_POINT('Origin',(0.,-0.05953,0.));
#19550=CARTESIAN_POINT('',(1.08212377959455,-0.05953,0.303251606722892));
#19551=CARTESIAN_POINT('Ctrl Pts',(1.08212377959455,-0.0595300000000001,
-0.303251606722892));
#19552=CARTESIAN_POINT('Ctrl Pts',(1.0830271513892,-0.0762225747374255,
-0.300028012588062));
#19553=CARTESIAN_POINT('Ctrl Pts',(1.08431331394788,-0.0928409665394228,
-0.2953917518996));
#19554=CARTESIAN_POINT('Ctrl Pts',(1.08940878963422,-0.144299303100741,
-0.276273267473431));
#19555=CARTESIAN_POINT('Ctrl Pts',(1.09443784939331,-0.177024326825049,
-0.256354979351213));
#19556=CARTESIAN_POINT('Ctrl Pts',(1.10373487993589,-0.227269801620064,
-0.212533521233765));
#19557=CARTESIAN_POINT('Ctrl Pts',(1.10909715583869,-0.251265615809407,
-0.183354415742157));
#19558=CARTESIAN_POINT('Ctrl Pts',(1.1160463456491,-0.279889827963178,-0.133783682657561));
#19559=CARTESIAN_POINT('Ctrl Pts',(1.11894887330541,-0.290879136862659,
-0.107881990270302));
#19560=CARTESIAN_POINT('Ctrl Pts',(1.12284346704144,-0.305251990234488,
-0.0539226701638766));
#19561=CARTESIAN_POINT('Ctrl Pts',(1.123812,-0.308638795020976,-0.025864214957475));
#19562=CARTESIAN_POINT('Ctrl Pts',(1.123812,-0.308638795020976,0.025864214957475));
#19563=CARTESIAN_POINT('Ctrl Pts',(1.12284346704144,-0.305251990234488,
0.0539226701638766));
#19564=CARTESIAN_POINT('Ctrl Pts',(1.11894887330541,-0.290879136862659,
0.107881990270302));
#19565=CARTESIAN_POINT('Ctrl Pts',(1.1160463456491,-0.279889827963178,0.133783682657561));
#19566=CARTESIAN_POINT('Ctrl Pts',(1.10909715583869,-0.251265615809407,
0.183354415742157));
#19567=CARTESIAN_POINT('Ctrl Pts',(1.10373487993589,-0.227269801620064,
0.212533521233765));
#19568=CARTESIAN_POINT('Ctrl Pts',(1.09443784939331,-0.177024326825049,
0.256354979351213));
#19569=CARTESIAN_POINT('Ctrl Pts',(1.08940878963422,-0.144299303100741,
0.276273267473431));
#19570=CARTESIAN_POINT('Ctrl Pts',(1.08431331394788,-0.0928409665394228,
0.2953917518996));
#19571=CARTESIAN_POINT('Ctrl Pts',(1.0830271513892,-0.0762225747374255,
0.300028012588062));
#19572=CARTESIAN_POINT('Ctrl Pts',(1.08212377959455,-0.0595300000000001,
0.303251606722892));
#19573=CARTESIAN_POINT('Origin',(0.,-0.05953,0.));
#19574=CARTESIAN_POINT('Origin',(0.,-0.05953,0.));
#19575=CARTESIAN_POINT('',(0.0589974094846122,-0.05953,1.07456964270265));
#19576=CARTESIAN_POINT('Origin',(0.,-0.05953,0.));
#19577=CARTESIAN_POINT('Origin',(-0.244773027351946,-0.05953,1.07242070340001));
#19578=CARTESIAN_POINT('Origin',(-0.244773027351946,0.,1.07242070340001));
#19579=CARTESIAN_POINT('',(-0.519393123750572,-0.05953,0.942555777842682));
#19580=CARTESIAN_POINT('Ctrl Pts',(-0.519393123750572,-0.05953,0.942555777842682));
#19581=CARTESIAN_POINT('Ctrl Pts',(-0.513714466572041,-0.0925528133349865,
0.945684988399766));
#19582=CARTESIAN_POINT('Ctrl Pts',(-0.503136848051455,-0.124911173756694,
0.951483858396181));
#19583=CARTESIAN_POINT('Ctrl Pts',(-0.47593627990192,-0.177924977804098,
0.965323333309091));
#19584=CARTESIAN_POINT('Ctrl Pts',(-0.460931856495794,-0.199697230012983,
0.972669835243841));
#19585=CARTESIAN_POINT('Ctrl Pts',(-0.426157505475872,-0.237895043532788,
0.988400002689705));
#19586=CARTESIAN_POINT('Ctrl Pts',(-0.406380688682952,-0.254319232363049,
0.996771768218699));
#19587=CARTESIAN_POINT('Ctrl Pts',(-0.364750145543744,-0.28018331644634,
1.01272583306292));
#19588=CARTESIAN_POINT('Ctrl Pts',(-0.340838910881557,-0.29104845371857,
1.02112815447116));
#19589=CARTESIAN_POINT('Ctrl Pts',(-0.290495481564827,-0.30527573347708,
1.036574285215));
#19590=CARTESIAN_POINT('Ctrl Pts',(-0.264056468041074,-0.308638795020976,
1.04359501395068));
#19591=CARTESIAN_POINT('Ctrl Pts',(-0.214892249704082,-0.308638795020976,
1.05481642595959));
#19592=CARTESIAN_POINT('Ctrl Pts',(-0.188025341585962,-0.30527573347708,
1.05996242598502));
#19593=CARTESIAN_POINT('Ctrl Pts',(-0.135965654106109,-0.29104845371857,
1.06788913840721));
#19594=CARTESIAN_POINT('Ctrl Pts',(-0.110776745452494,-0.28018331644634,
1.07069360430242));
#19595=CARTESIAN_POINT('Ctrl Pts',(-0.0663467128214646,-0.254319232363049,
1.07438230428002));
#19596=CARTESIAN_POINT('Ctrl Pts',(-0.0448960436540983,-0.237895043532788,
1.07542044338697));
#19597=CARTESIAN_POINT('Ctrl Pts',(-0.00674037211528124,-0.199697230012983,
1.07633607767727));
#19598=CARTESIAN_POINT('Ctrl Pts',(0.00996567398334777,-0.177924977804098,
1.07622728347683));
#19599=CARTESIAN_POINT('Ctrl Pts',(0.0404772621979741,-0.124911173756694,
1.07556023164702));
#19600=CARTESIAN_POINT('Ctrl Pts',(0.0525234025782719,-0.0925528133349865,
1.07492508698591));
#19601=CARTESIAN_POINT('Ctrl Pts',(0.0589974094846124,-0.05953,1.07456964270265));
#19602=CARTESIAN_POINT('Origin',(-0.244773027351946,-0.05953,1.07242070340001));
#19603=CARTESIAN_POINT('Origin',(0.,-0.05953,0.));
#19604=CARTESIAN_POINT('',(-0.803348093619616,-0.05953,0.716109245731214));
#19605=CARTESIAN_POINT('Origin',(0.,-0.05953,0.));
#19606=CARTESIAN_POINT('Origin',(-0.991065754692661,-0.05953,0.477272113029314));
#19607=CARTESIAN_POINT('Origin',(-0.991065754692661,0.,0.477272113029314));
#19608=CARTESIAN_POINT('',(-1.06075609691358,-0.05953,0.181596019242328));
#19609=CARTESIAN_POINT('Ctrl Pts',(-1.06075609691358,-0.05953,0.181596019242328));
#19610=CARTESIAN_POINT('Ctrl Pts',(-1.05966202740332,-0.0925528133349865,
0.187986803072856));
#19611=CARTESIAN_POINT('Ctrl Pts',(-1.05760072925372,-0.124911173756694,
0.199872254546857));
#19612=CARTESIAN_POINT('Ctrl Pts',(-1.05146158959546,-0.177924977804098,
0.22976728653846));
#19613=CARTESIAN_POINT('Ctrl Pts',(-1.04785021111757,-0.199697230012983,
0.246078686169301));
#19614=CARTESIAN_POINT('Ctrl Pts',(-1.03846709802406,-0.237895043532788,
0.283073967563097));
#19615=CARTESIAN_POINT('Ctrl Pts',(-1.03268176429485,-0.254319232363049,
0.303755815985685));
#19616=CARTESIAN_POINT('Ctrl Pts',(-1.01919893537026,-0.28018331644634,
0.346251081972725));
#19617=CARTESIAN_POINT('Ctrl Pts',(-1.01085972381132,-0.29104845371857,
0.370184399726282));
#19618=CARTESIAN_POINT('Ctrl Pts',(-0.99154738033959,-0.30527573347708,
0.419174982698463));
#19619=CARTESIAN_POINT('Ctrl Pts',(-0.980551951791748,-0.308638795020976,
0.444223188605045));
#19620=CARTESIAN_POINT('Ctrl Pts',(-0.958671816228589,-0.308638795020976,
0.489657758261848));
#19621=CARTESIAN_POINT('Ctrl Pts',(-0.945943877838127,-0.30527573347708,
0.51387163140139));
#19622=CARTESIAN_POINT('Ctrl Pts',(-0.91968254693063,-0.29104845371857,
0.559515758398093));
#19623=CARTESIAN_POINT('Ctrl Pts',(-0.906170138993533,-0.28018331644634,
0.580957796077825));
#19624=CARTESIAN_POINT('Ctrl Pts',(-0.8813524085237,-0.254319232363049,
0.617994461173994));
#19625=CARTESIAN_POINT('Ctrl Pts',(-0.868789784891799,-0.237895043532788,
0.635412538795143));
#19626=CARTESIAN_POINT('Ctrl Pts',(-0.845715984518854,-0.199697230012983,
0.66581473268113));
#19627=CARTESIAN_POINT('Ctrl Pts',(-0.835214876415962,-0.177924977804098,
0.678808213394124));
#19628=CARTESIAN_POINT('Ctrl Pts',(-0.815669690204649,-0.124911173756694,
0.702247233627224));
#19629=CARTESIAN_POINT('Ctrl Pts',(-0.807662468433796,-0.0925528133349865,
0.711269279199861));
#19630=CARTESIAN_POINT('Ctrl Pts',(-0.803348093619616,-0.05953,0.716109245731214));
#19631=CARTESIAN_POINT('Origin',(-0.991065754692661,-0.05953,0.477272113029314));
#19632=CARTESIAN_POINT('Origin',(0.,-0.05953,0.));
#19633=CARTESIAN_POINT('',(-1.076188,-0.05953,1.31795018948079E-16));
#19634=CARTESIAN_POINT('Origin',(0.,-0.05953,0.));
#19635=CARTESIAN_POINT('',(-1.06075609691358,-0.05953,-0.181596019242328));
#19636=CARTESIAN_POINT('Origin',(0.,-0.05953,0.));
#19637=CARTESIAN_POINT('Origin',(-0.991065754692661,-0.05953,-0.477272113029314));
#19638=CARTESIAN_POINT('Origin',(-0.991065754692661,0.,-0.477272113029314));
#19639=CARTESIAN_POINT('',(-0.803348093619616,-0.05953,-0.716109245731215));
#19640=CARTESIAN_POINT('Ctrl Pts',(-0.803348093619616,-0.05953,-0.716109245731215));
#19641=CARTESIAN_POINT('Ctrl Pts',(-0.807662468433795,-0.0925528133349865,
-0.711269279199862));
#19642=CARTESIAN_POINT('Ctrl Pts',(-0.815669690204649,-0.124911173756694,
-0.702247233627224));
#19643=CARTESIAN_POINT('Ctrl Pts',(-0.835214876415962,-0.177924977804098,
-0.678808213394124));
#19644=CARTESIAN_POINT('Ctrl Pts',(-0.845715984518854,-0.199697230012983,
-0.66581473268113));
#19645=CARTESIAN_POINT('Ctrl Pts',(-0.868789784891799,-0.237895043532788,
-0.635412538795143));
#19646=CARTESIAN_POINT('Ctrl Pts',(-0.8813524085237,-0.254319232363049,
-0.617994461173994));
#19647=CARTESIAN_POINT('Ctrl Pts',(-0.906170138993533,-0.28018331644634,
-0.580957796077826));
#19648=CARTESIAN_POINT('Ctrl Pts',(-0.91968254693063,-0.29104845371857,
-0.559515758398093));
#19649=CARTESIAN_POINT('Ctrl Pts',(-0.945943877838127,-0.30527573347708,
-0.51387163140139));
#19650=CARTESIAN_POINT('Ctrl Pts',(-0.958671816228589,-0.308638795020976,
-0.489657758261848));
#19651=CARTESIAN_POINT('Ctrl Pts',(-0.980551951791748,-0.308638795020976,
-0.444223188605045));
#19652=CARTESIAN_POINT('Ctrl Pts',(-0.99154738033959,-0.30527573347708,
-0.419174982698463));
#19653=CARTESIAN_POINT('Ctrl Pts',(-1.01085972381132,-0.29104845371857,
-0.370184399726282));
#19654=CARTESIAN_POINT('Ctrl Pts',(-1.01919893537026,-0.28018331644634,
-0.346251081972725));
#19655=CARTESIAN_POINT('Ctrl Pts',(-1.03268176429485,-0.254319232363049,
-0.303755815985685));
#19656=CARTESIAN_POINT('Ctrl Pts',(-1.03846709802406,-0.237895043532788,
-0.283073967563097));
#19657=CARTESIAN_POINT('Ctrl Pts',(-1.04785021111757,-0.199697230012983,
-0.246078686169302));
#19658=CARTESIAN_POINT('Ctrl Pts',(-1.05146158959546,-0.177924977804098,
-0.229767286538461));
#19659=CARTESIAN_POINT('Ctrl Pts',(-1.05760072925372,-0.124911173756694,
-0.199872254546858));
#19660=CARTESIAN_POINT('Ctrl Pts',(-1.05966202740332,-0.0925528133349864,
-0.187986803072857));
#19661=CARTESIAN_POINT('Ctrl Pts',(-1.06075609691358,-0.05953,-0.181596019242328));
#19662=CARTESIAN_POINT('Origin',(-0.991065754692661,-0.05953,-0.477272113029314));
#19663=CARTESIAN_POINT('Origin',(0.,-0.05953,0.));
#19664=CARTESIAN_POINT('',(-0.519393123750572,-0.05953,-0.942555777842682));
#19665=CARTESIAN_POINT('Origin',(0.,-0.05953,0.));
#19666=CARTESIAN_POINT('Origin',(-0.244773027351946,-0.05953,-1.07242070340001));
#19667=CARTESIAN_POINT('Origin',(-0.244773027351946,0.,-1.07242070340001));
#19668=CARTESIAN_POINT('',(0.0589974094846125,-0.05953,-1.07456964270265));
#19669=CARTESIAN_POINT('Ctrl Pts',(0.0589974094846127,-0.05953,-1.07456964270265));
#19670=CARTESIAN_POINT('Ctrl Pts',(0.0525234025782722,-0.0925528133349865,
-1.07492508698591));
#19671=CARTESIAN_POINT('Ctrl Pts',(0.0404772621979744,-0.124911173756694,
-1.07556023164702));
#19672=CARTESIAN_POINT('Ctrl Pts',(0.0099656739833481,-0.177924977804098,
-1.07622728347683));
#19673=CARTESIAN_POINT('Ctrl Pts',(-0.00674037211528096,-0.199697230012983,
-1.07633607767727));
#19674=CARTESIAN_POINT('Ctrl Pts',(-0.044896043654098,-0.237895043532788,
-1.07542044338697));
#19675=CARTESIAN_POINT('Ctrl Pts',(-0.0663467128214644,-0.254319232363049,
-1.07438230428002));
#19676=CARTESIAN_POINT('Ctrl Pts',(-0.110776745452493,-0.28018331644634,
-1.07069360430242));
#19677=CARTESIAN_POINT('Ctrl Pts',(-0.135965654106109,-0.29104845371857,
-1.06788913840721));
#19678=CARTESIAN_POINT('Ctrl Pts',(-0.188025341585962,-0.30527573347708,
-1.05996242598502));
#19679=CARTESIAN_POINT('Ctrl Pts',(-0.214892249704082,-0.308638795020976,
-1.05481642595959));
#19680=CARTESIAN_POINT('Ctrl Pts',(-0.264056468041074,-0.308638795020976,
-1.04359501395068));
#19681=CARTESIAN_POINT('Ctrl Pts',(-0.290495481564827,-0.30527573347708,
-1.036574285215));
#19682=CARTESIAN_POINT('Ctrl Pts',(-0.340838910881557,-0.291048453718569,
-1.02112815447116));
#19683=CARTESIAN_POINT('Ctrl Pts',(-0.364750145543744,-0.28018331644634,
-1.01272583306292));
#19684=CARTESIAN_POINT('Ctrl Pts',(-0.406380688682952,-0.254319232363049,
-0.996771768218699));
#19685=CARTESIAN_POINT('Ctrl Pts',(-0.426157505475872,-0.237895043532788,
-0.988400002689705));
#19686=CARTESIAN_POINT('Ctrl Pts',(-0.460931856495794,-0.199697230012983,
-0.972669835243841));
#19687=CARTESIAN_POINT('Ctrl Pts',(-0.475936279901919,-0.177924977804098,
-0.965323333309091));
#19688=CARTESIAN_POINT('Ctrl Pts',(-0.503136848051454,-0.124911173756694,
-0.951483858396181));
#19689=CARTESIAN_POINT('Ctrl Pts',(-0.513714466572041,-0.0925528133349865,
-0.945684988399766));
#19690=CARTESIAN_POINT('Ctrl Pts',(-0.519393123750572,-0.05953,-0.942555777842682));
#19691=CARTESIAN_POINT('Origin',(-0.244773027351946,-0.05953,-1.07242070340001));
#19692=CARTESIAN_POINT('Origin',(0.,-0.05953,0.));
#19693=CARTESIAN_POINT('',(0.413083465285518,-0.05953,-0.993751811093549));
#19694=CARTESIAN_POINT('Origin',(0.,-0.05953,0.));
#19695=CARTESIAN_POINT('Origin',(0.685838782044607,-0.05953,-0.860014630714833));
#19696=CARTESIAN_POINT('Origin',(0.685838782044607,0.,-0.860014630714833));
#19697=CARTESIAN_POINT('',(0.876916659919095,-0.05953,-0.623857181492959));
#19698=CARTESIAN_POINT('Ctrl Pts',(0.876916659919095,-0.05953,-0.623857181492958));
#19699=CARTESIAN_POINT('Ctrl Pts',(0.873158080166742,-0.0925528133349865,
-0.62914037979579));
#19700=CARTESIAN_POINT('Ctrl Pts',(0.866144010579847,-0.124911173756694,
-0.638954437806245));
#19701=CARTESIAN_POINT('Ctrl Pts',(0.847641868610495,-0.177924977804098,
-0.663225258065736));
#19702=CARTESIAN_POINT('Ctrl Pts',(0.837310877969633,-0.199697230012983,
-0.676354402927683));
#19703=CARTESIAN_POINT('Ctrl Pts',(0.81280533416753,-0.237895043532788,
-0.705614819529209));
#19704=CARTESIAN_POINT('Ctrl Pts',(0.798619410861634,-0.254319232363049,
-0.721738358858166));
#19705=CARTESIAN_POINT('Ctrl Pts',(0.768033796848072,-0.28018331644634,
-0.754175290318038));
#19706=CARTESIAN_POINT('Ctrl Pts',(0.750136149454208,-0.29104845371857,
-0.772120216227122));
#19707=CARTESIAN_POINT('Ctrl Pts',(0.711480111898423,-0.30527573347708,
-0.807879894508811));
#19708=CARTESIAN_POINT('Ctrl Pts',(0.690705563850638,-0.308638795020976,
-0.825676810575913));
#19709=CARTESIAN_POINT('Ctrl Pts',(0.651278921914856,-0.308638795020976,
-0.857118508332695));
#19710=CARTESIAN_POINT('Ctrl Pts',(0.629305439856167,-0.30527573347708,
-0.873412008702649));
#19711=CARTESIAN_POINT('Ctrl Pts',(0.585840553788742,-0.29104845371857,
-0.903141581680914));
#19712=CARTESIAN_POINT('Ctrl Pts',(0.564362943424239,-0.28018331644634,
-0.916597376014514));
#19713=CARTESIAN_POINT('Ctrl Pts',(0.525933334162556,-0.254319232363049,
-0.939198248544427));
#19714=CARTESIAN_POINT('Ctrl Pts',(0.507057380724533,-0.237895043532788,
-0.949440676105255));
#19715=CARTESIAN_POINT('Ctrl Pts',(0.473077587363686,-0.199697230012983,
-0.966820759530997));
#19716=CARTESIAN_POINT('Ctrl Pts',(0.457978755888596,-0.177924977804098,
-0.973971221090534));
#19717=CARTESIAN_POINT('Ctrl Pts',(0.430199341854858,-0.124911173756694,
-0.986608710139579));
#19718=CARTESIAN_POINT('Ctrl Pts',(0.419070565453384,-0.0925528133349865,
-0.991263089003441));
#19719=CARTESIAN_POINT('Ctrl Pts',(0.413083465285518,-0.05953,-0.993751811093549));
#19720=CARTESIAN_POINT('Origin',(0.685838782044607,-0.05953,-0.860014630714833));
#19721=CARTESIAN_POINT('Origin',(0.,-0.208355,0.));
#19722=CARTESIAN_POINT('',(-1.076188,-0.35718,1.31795018948079E-16));
#19723=CARTESIAN_POINT('Origin',(0.,-0.35718,0.));
#19724=CARTESIAN_POINT('',(-1.076188,-0.208355,1.31795018948079E-16));
#19725=CARTESIAN_POINT('',(1.03449977959455,-0.05953,0.296632461748266));
#19726=CARTESIAN_POINT('Origin',(0.,-0.05953,0.));
#19727=CARTESIAN_POINT('',(1.03449977959455,-0.05953,-0.296632461748266));
#19728=CARTESIAN_POINT('Ctrl Pts',(1.03449977959455,-0.05953,0.296632461748267));
#19729=CARTESIAN_POINT('Ctrl Pts',(1.03628691421076,-0.0925528133349865,
0.290399865505497));
#19730=CARTESIAN_POINT('Ctrl Pts',(1.03958665287714,-0.124911173756694,
0.278797079997872));
#19731=CARTESIAN_POINT('Ctrl Pts',(1.0470264474309,-0.177924977804098,0.249198913998601));
#19732=CARTESIAN_POINT('Ctrl Pts',(1.05084995891418,-0.199697230012983,
0.232935932341942));
#19733=CARTESIAN_POINT('Ctrl Pts',(1.05844771715377,-0.237895043532788,
0.195533155353269));
#19734=CARTESIAN_POINT('Ctrl Pts',(1.06220882929878,-0.254319232363049,
0.17438929156337));
#19735=CARTESIAN_POINT('Ctrl Pts',(1.06849922508772,-0.28018331644634,0.130252399648131));
#19736=CARTESIAN_POINT('Ctrl Pts',(1.07137013248666,-0.29104845371857,0.105070977154072));
#19737=CARTESIAN_POINT('Ctrl Pts',(1.07522652957392,-0.30527573347708,0.0525526752791107));
#19738=CARTESIAN_POINT('Ctrl Pts',(1.076188,-0.308638795020976,0.025214283908933));
#19739=CARTESIAN_POINT('Ctrl Pts',(1.076188,-0.308638795020976,-0.025214283908933));
#19740=CARTESIAN_POINT('Ctrl Pts',(1.07522652957392,-0.30527573347708,-0.0525526752791107));
#19741=CARTESIAN_POINT('Ctrl Pts',(1.07137013248666,-0.29104845371857,-0.105070977154072));
#19742=CARTESIAN_POINT('Ctrl Pts',(1.06849922508772,-0.28018331644634,-0.130252399648131));
#19743=CARTESIAN_POINT('Ctrl Pts',(1.06220882929878,-0.254319232363049,
-0.17438929156337));
#19744=CARTESIAN_POINT('Ctrl Pts',(1.05844771715377,-0.237895043532788,
-0.195533155353269));
#19745=CARTESIAN_POINT('Ctrl Pts',(1.05084995891418,-0.199697230012983,
-0.232935932341942));
#19746=CARTESIAN_POINT('Ctrl Pts',(1.0470264474309,-0.177924977804098,-0.249198913998601));
#19747=CARTESIAN_POINT('Ctrl Pts',(1.03958665287714,-0.124911173756694,
-0.278797079997872));
#19748=CARTESIAN_POINT('Ctrl Pts',(1.03628691421076,-0.0925528133349865,
-0.290399865505497));
#19749=CARTESIAN_POINT('Ctrl Pts',(1.03449977959455,-0.05953,-0.296632461748267));
#19750=CARTESIAN_POINT('Origin',(0.,-0.05953,0.));
#19751=CARTESIAN_POINT('Origin',(0.,-0.05953,0.));
#19752=CARTESIAN_POINT('Origin',(1.1,-0.05953,0.));
#19753=CARTESIAN_POINT('Origin',(1.1,0.,0.));
#19754=CARTESIAN_POINT('Origin',(1.1,-0.05953,0.));
#19755=CARTESIAN_POINT('Origin',(0.,-0.35718,0.));
#19756=CARTESIAN_POINT('Origin',(0.,-0.05953,0.));
#33893=UNCERTAINTY_MEASURE_WITH_UNIT(LENGTH_MEASURE(0.001),#33982,
'DISTANCE_ACCURACY_VALUE',
'Maximum model space distance between geometric entities at asserted c
onnectivities');
#33929=UNCERTAINTY_MEASURE_WITH_UNIT(LENGTH_MEASURE(0.001),#33982,
'DISTANCE_ACCURACY_VALUE',
'Maximum model space distance between geometric entities at asserted c
onnectivities');
#33945=(
GEOMETRIC_REPRESENTATION_CONTEXT(3)
GLOBAL_UNCERTAINTY_ASSIGNED_CONTEXT((#33893))
GLOBAL_UNIT_ASSIGNED_CONTEXT((#33982,#33984,#33985))
REPRESENTATION_CONTEXT('','3D')
);
#33981=(
GEOMETRIC_REPRESENTATION_CONTEXT(3)
GLOBAL_UNCERTAINTY_ASSIGNED_CONTEXT((#33929))
GLOBAL_UNIT_ASSIGNED_CONTEXT((#33982,#33984,#33985))
REPRESENTATION_CONTEXT('','3D')
);
#33982=(
LENGTH_UNIT()
NAMED_UNIT(*)
SI_UNIT(.CENTI.,.METRE.)
);
#33984=(
NAMED_UNIT(*)
PLANE_ANGLE_UNIT()
SI_UNIT($,.RADIAN.)
);
#33985=(
NAMED_UNIT(*)
SI_UNIT($,.STERADIAN.)
SOLID_ANGLE_UNIT()
);
#34001=SHAPE_DEFINITION_REPRESENTATION(#34052,#34197);
#34052=PRODUCT_DEFINITION_SHAPE('',$,#34249);
#34197=SHAPE_REPRESENTATION('',(#13927),#33945);
#34233=PRODUCT_DEFINITION_CONTEXT('part definition',#34388,'design');
#34249=PRODUCT_DEFINITION('Cage','Cage',#34300,#34233);
#34300=PRODUCT_DEFINITION_FORMATION('',$,#34405);
#34388=APPLICATION_CONTEXT(
'Core Data for Automotive Mechanical Design Process');
#34389=PRODUCT_CONTEXT('part definition',#34388,'mechanical');
#34405=PRODUCT('Cage','Cage','Cage',(#34389));
#34511=COLOUR_RGB('Grey',0.48,0.52,0.57);
#34512=FILL_AREA_STYLE_COLOUR('',#34511);
#34513=FILL_AREA_STYLE('',(#34512));
#34514=SURFACE_STYLE_FILL_AREA(#34513);
#34515=SURFACE_SIDE_STYLE('',(#34514));
#34516=SURFACE_STYLE_USAGE(.BOTH.,#34515);
#34517=PRESENTATION_STYLE_ASSIGNMENT((#34516));
ENDSEC;
END-ISO-10303-21;
